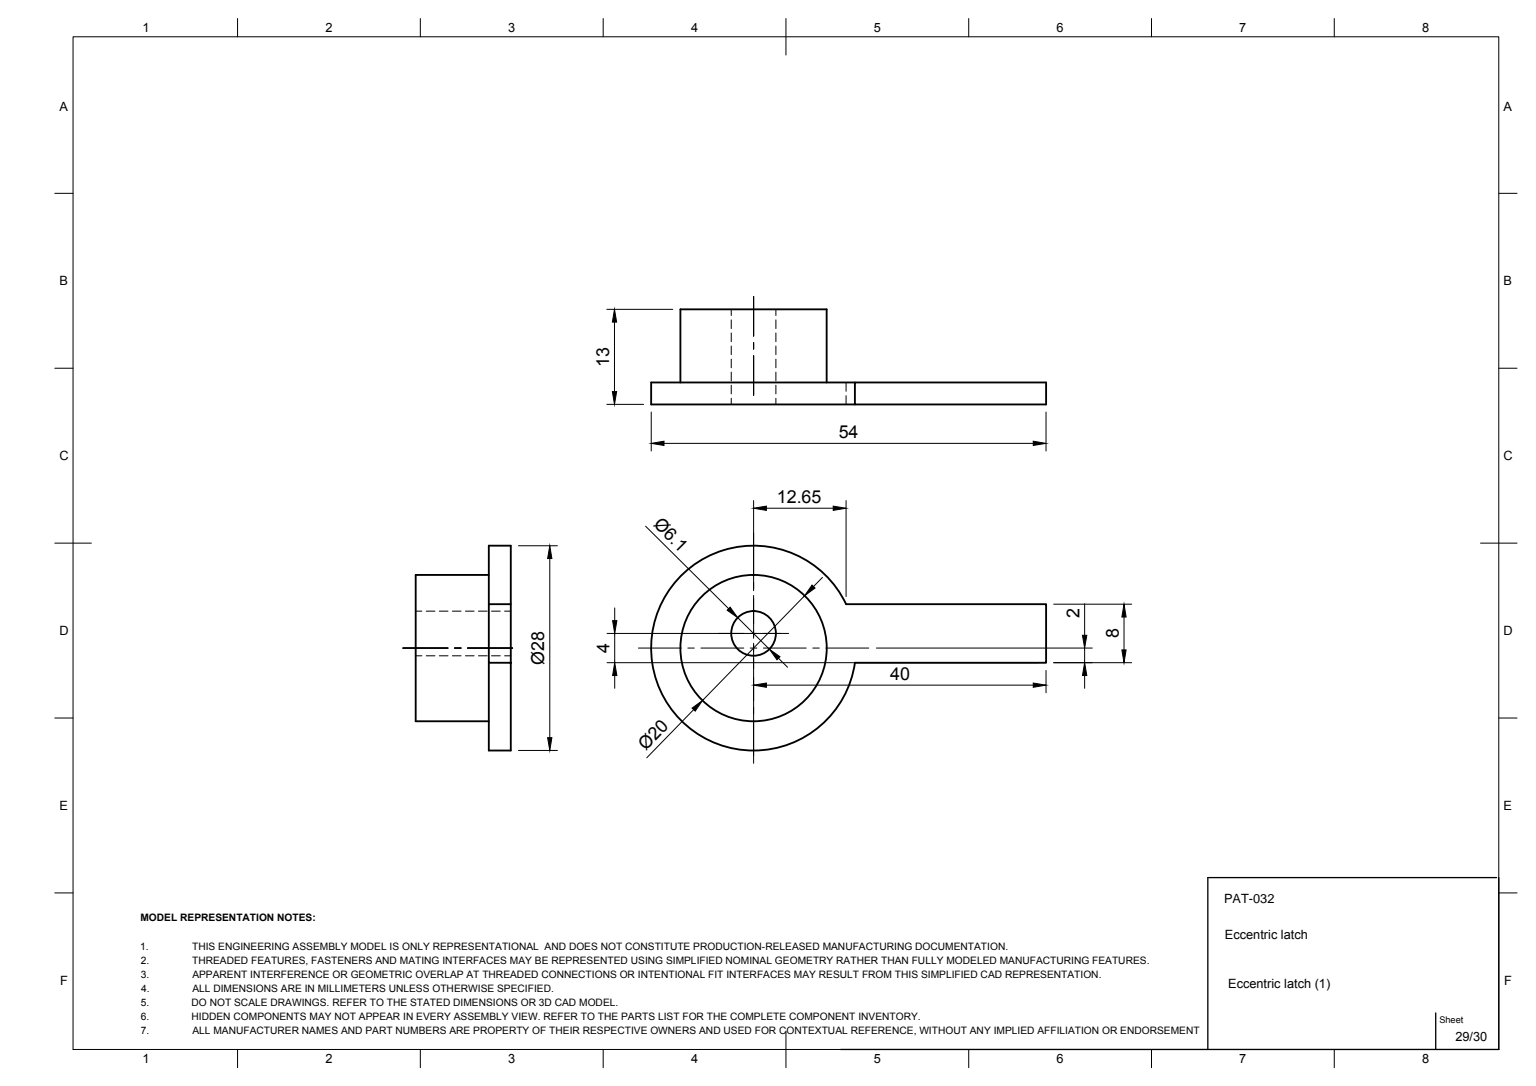
ISO-10303-21;
HEADER;
/* Generated by software containing ST-Developer
 * from STEP Tools, Inc. (www.steptools.com) 
 */

FILE_DESCRIPTION(
/* description */ ('Drill jig with bushing plate'),
/* implementation_level */ '2;1');

FILE_NAME(
/* name */ 'Eccentric latch.step',
/* time_stamp */ '2026-10-27T10:51:08-07:00',
/* author */ (''),
/* organization */ (''),
/* preprocessor_version */ 'ST-DEVELOPER v20.2',
/* originating_system */ 'Autodesk Translation Framework v15.17.0.0',
/* authorisation */ '');

FILE_SCHEMA (('AUTOMOTIVE_DESIGN { 1 0 10303 214 3 1 1 }'));
ENDSEC;

DATA;
#10=MECHANICAL_DESIGN_GEOMETRIC_PRESENTATION_REPRESENTATION('',(#245),#6638);
#197=SHAPE_REPRESENTATION_RELATIONSHIP('SRR','None',#6763,#221);
#221=ADVANCED_BREP_SHAPE_REPRESENTATION('',(#267),#6636);
#245=STYLED_ITEM('',(#6936),#267);
#267=MANIFOLD_SOLID_BREP('Body1',#3614);
#367=FACE_BOUND('',#1020,.T.);
#368=FACE_BOUND('',#1022,.T.);
#369=FACE_BOUND('',#1026,.T.);
#493=PLANE('',#4306);
#494=PLANE('',#4307);
#495=PLANE('',#4308);
#496=PLANE('',#4309);
#497=PLANE('',#4311);
#498=PLANE('',#4317);
#703=FACE_OUTER_BOUND('',#1015,.T.);
#704=FACE_OUTER_BOUND('',#1016,.T.);
#705=FACE_OUTER_BOUND('',#1017,.T.);
#706=FACE_OUTER_BOUND('',#1018,.T.);
#707=FACE_OUTER_BOUND('',#1019,.T.);
#708=FACE_OUTER_BOUND('',#1021,.T.);
#709=FACE_OUTER_BOUND('',#1023,.T.);
#710=FACE_OUTER_BOUND('',#1024,.T.);
#711=FACE_OUTER_BOUND('',#1025,.T.);
#1015=EDGE_LOOP('',(#3257,#3258,#3259,#3260));
#1016=EDGE_LOOP('',(#3261,#3262,#3263,#3264));
#1017=EDGE_LOOP('',(#3265,#3266,#3267,#3268));
#1018=EDGE_LOOP('',(#3269,#3270,#3271,#3272));
#1019=EDGE_LOOP('',(#3273,#3274,#3275,#3276));
#1020=EDGE_LOOP('',(#3277));
#1021=EDGE_LOOP('',(#3278,#3279,#3280,#3281));
#1022=EDGE_LOOP('',(#3282));
#1023=EDGE_LOOP('',(#3283,#3284,#3285,#3286));
#1024=EDGE_LOOP('',(#3287,#3288,#3289,#3290));
#1025=EDGE_LOOP('',(#3291));
#1026=EDGE_LOOP('',(#3292));
#1278=LINE('',#6532,#1539);
#1279=LINE('',#6537,#1540);
#1280=LINE('',#6539,#1541);
#1281=LINE('',#6541,#1542);
#1282=LINE('',#6542,#1543);
#1283=LINE('',#6545,#1544);
#1284=LINE('',#6547,#1545);
#1285=LINE('',#6548,#1546);
#1286=LINE('',#6552,#1547);
#1287=LINE('',#6553,#1548);
#1288=LINE('',#6554,#1549);
#1289=LINE('',#6564,#1550);
#1539=VECTOR('',#5425,0.305);
#1540=VECTOR('',#5430,1.);
#1541=VECTOR('',#5431,1.);
#1542=VECTOR('',#5432,1.);
#1543=VECTOR('',#5433,1.);
#1544=VECTOR('',#5436,1.);
#1545=VECTOR('',#5437,1.);
#1546=VECTOR('',#5438,1.);
#1547=VECTOR('',#5441,1.);
#1548=VECTOR('',#5442,1.);
#1549=VECTOR('',#5443,1.);
#1550=VECTOR('',#5458,1.);
#1712=CIRCLE('',#4304,0.305);
#1713=CIRCLE('',#4305,0.305);
#1714=CIRCLE('',#4310,1.4);
#1715=CIRCLE('',#4312,1.4);
#1716=CIRCLE('',#4313,1.);
#1717=CIRCLE('',#4316,1.);
#1992=VERTEX_POINT('',#6529);
#1993=VERTEX_POINT('',#6531);
#1994=VERTEX_POINT('',#6535);
#1995=VERTEX_POINT('',#6536);
#1996=VERTEX_POINT('',#6538);
#1997=VERTEX_POINT('',#6540);
#1998=VERTEX_POINT('',#6544);
#1999=VERTEX_POINT('',#6546);
#2000=VERTEX_POINT('',#6550);
#2001=VERTEX_POINT('',#6551);
#2002=VERTEX_POINT('',#6559);
#2003=VERTEX_POINT('',#6563);
#2416=EDGE_CURVE('',#1992,#1992,#1712,.T.);
#2417=EDGE_CURVE('',#1992,#1993,#1278,.T.);
#2418=EDGE_CURVE('',#1993,#1993,#1713,.T.);
#2419=EDGE_CURVE('',#1994,#1995,#1279,.T.);
#2420=EDGE_CURVE('',#1994,#1996,#1280,.T.);
#2421=EDGE_CURVE('',#1996,#1997,#1281,.T.);
#2422=EDGE_CURVE('',#1995,#1997,#1282,.T.);
#2423=EDGE_CURVE('',#1996,#1998,#1283,.T.);
#2424=EDGE_CURVE('',#1998,#1999,#1284,.T.);
#2425=EDGE_CURVE('',#1997,#1999,#1285,.T.);
#2426=EDGE_CURVE('',#2000,#2001,#1286,.T.);
#2427=EDGE_CURVE('',#1999,#2000,#1287,.T.);
#2428=EDGE_CURVE('',#1998,#2001,#1288,.T.);
#2429=EDGE_CURVE('',#2000,#1995,#1714,.T.);
#2430=EDGE_CURVE('',#2001,#1994,#1715,.T.);
#2431=EDGE_CURVE('',#2002,#2002,#1716,.T.);
#2432=EDGE_CURVE('',#2002,#2003,#1289,.T.);
#2433=EDGE_CURVE('',#2003,#2003,#1717,.T.);
#3257=ORIENTED_EDGE('',*,*,#2416,.F.);
#3258=ORIENTED_EDGE('',*,*,#2417,.T.);
#3259=ORIENTED_EDGE('',*,*,#2418,.F.);
#3260=ORIENTED_EDGE('',*,*,#2417,.F.);
#3261=ORIENTED_EDGE('',*,*,#2419,.F.);
#3262=ORIENTED_EDGE('',*,*,#2420,.T.);
#3263=ORIENTED_EDGE('',*,*,#2421,.T.);
#3264=ORIENTED_EDGE('',*,*,#2422,.F.);
#3265=ORIENTED_EDGE('',*,*,#2423,.T.);
#3266=ORIENTED_EDGE('',*,*,#2424,.T.);
#3267=ORIENTED_EDGE('',*,*,#2425,.F.);
#3268=ORIENTED_EDGE('',*,*,#2421,.F.);
#3269=ORIENTED_EDGE('',*,*,#2426,.F.);
#3270=ORIENTED_EDGE('',*,*,#2427,.F.);
#3271=ORIENTED_EDGE('',*,*,#2424,.F.);
#3272=ORIENTED_EDGE('',*,*,#2428,.T.);
#3273=ORIENTED_EDGE('',*,*,#2429,.T.);
#3274=ORIENTED_EDGE('',*,*,#2422,.T.);
#3275=ORIENTED_EDGE('',*,*,#2425,.T.);
#3276=ORIENTED_EDGE('',*,*,#2427,.T.);
#3277=ORIENTED_EDGE('',*,*,#2418,.T.);
#3278=ORIENTED_EDGE('',*,*,#2430,.F.);
#3279=ORIENTED_EDGE('',*,*,#2428,.F.);
#3280=ORIENTED_EDGE('',*,*,#2423,.F.);
#3281=ORIENTED_EDGE('',*,*,#2420,.F.);
#3282=ORIENTED_EDGE('',*,*,#2431,.T.);
#3283=ORIENTED_EDGE('',*,*,#2419,.T.);
#3284=ORIENTED_EDGE('',*,*,#2429,.F.);
#3285=ORIENTED_EDGE('',*,*,#2426,.T.);
#3286=ORIENTED_EDGE('',*,*,#2430,.T.);
#3287=ORIENTED_EDGE('',*,*,#2431,.F.);
#3288=ORIENTED_EDGE('',*,*,#2432,.T.);
#3289=ORIENTED_EDGE('',*,*,#2433,.T.);
#3290=ORIENTED_EDGE('',*,*,#2432,.F.);
#3291=ORIENTED_EDGE('',*,*,#2433,.F.);
#3292=ORIENTED_EDGE('',*,*,#2416,.T.);
#3372=CYLINDRICAL_SURFACE('',#4303,0.305);
#3373=CYLINDRICAL_SURFACE('',#4314,1.4);
#3374=CYLINDRICAL_SURFACE('',#4315,1.);
#3578=ADVANCED_FACE('',(#703),#3372,.F.);
#3579=ADVANCED_FACE('',(#704),#493,.T.);
#3580=ADVANCED_FACE('',(#705),#494,.T.);
#3581=ADVANCED_FACE('',(#706),#495,.T.);
#3582=ADVANCED_FACE('',(#707,#367),#496,.T.);
#3583=ADVANCED_FACE('',(#708,#368),#497,.F.);
#3584=ADVANCED_FACE('',(#709),#3373,.T.);
#3585=ADVANCED_FACE('',(#710),#3374,.T.);
#3586=ADVANCED_FACE('',(#711,#369),#498,.F.);
#3614=CLOSED_SHELL('',(#3578,#3579,#3580,#3581,#3582,#3583,#3584,#3585,
#3586));
#4302=AXIS2_PLACEMENT_3D('',#6527,#5419,#5420);
#4303=AXIS2_PLACEMENT_3D('',#6528,#5421,#5422);
#4304=AXIS2_PLACEMENT_3D('',#6530,#5423,#5424);
#4305=AXIS2_PLACEMENT_3D('',#6533,#5426,#5427);
#4306=AXIS2_PLACEMENT_3D('',#6534,#5428,#5429);
#4307=AXIS2_PLACEMENT_3D('',#6543,#5434,#5435);
#4308=AXIS2_PLACEMENT_3D('',#6549,#5439,#5440);
#4309=AXIS2_PLACEMENT_3D('',#6555,#5444,#5445);
#4310=AXIS2_PLACEMENT_3D('',#6556,#5446,#5447);
#4311=AXIS2_PLACEMENT_3D('',#6557,#5448,#5449);
#4312=AXIS2_PLACEMENT_3D('',#6558,#5450,#5451);
#4313=AXIS2_PLACEMENT_3D('',#6560,#5452,#5453);
#4314=AXIS2_PLACEMENT_3D('',#6561,#5454,#5455);
#4315=AXIS2_PLACEMENT_3D('',#6562,#5456,#5457);
#4316=AXIS2_PLACEMENT_3D('',#6565,#5459,#5460);
#4317=AXIS2_PLACEMENT_3D('',#6566,#5461,#5462);
#5419=DIRECTION('axis',(0.,0.,1.));
#5420=DIRECTION('refdir',(1.,0.,0.));
#5421=DIRECTION('center_axis',(0.,0.,1.));
#5422=DIRECTION('ref_axis',(1.,0.,0.));
#5423=DIRECTION('center_axis',(0.,0.,1.));
#5424=DIRECTION('ref_axis',(1.,0.,0.));
#5425=DIRECTION('',(0.,0.,1.));
#5426=DIRECTION('center_axis',(0.,0.,-1.));
#5427=DIRECTION('ref_axis',(1.,0.,0.));
#5428=DIRECTION('center_axis',(1.,0.,0.));
#5429=DIRECTION('ref_axis',(0.,1.,0.));
#5430=DIRECTION('',(0.,0.,1.));
#5431=DIRECTION('',(0.,1.,0.));
#5432=DIRECTION('',(0.,0.,1.));
#5433=DIRECTION('',(0.,1.,0.));
#5434=DIRECTION('center_axis',(0.,1.,0.));
#5435=DIRECTION('ref_axis',(-1.,0.,0.));
#5436=DIRECTION('',(-1.,0.,0.));
#5437=DIRECTION('',(0.,0.,1.));
#5438=DIRECTION('',(-1.,0.,0.));
#5439=DIRECTION('center_axis',(-1.,0.,0.));
#5440=DIRECTION('ref_axis',(0.,-1.,0.));
#5441=DIRECTION('',(0.,0.,-1.));
#5442=DIRECTION('',(0.,-1.,0.));
#5443=DIRECTION('',(0.,-1.,0.));
#5444=DIRECTION('center_axis',(0.,0.,1.));
#5445=DIRECTION('ref_axis',(1.,0.,0.));
#5446=DIRECTION('center_axis',(0.,0.,1.));
#5447=DIRECTION('ref_axis',(1.,0.,0.));
#5448=DIRECTION('center_axis',(0.,0.,1.));
#5449=DIRECTION('ref_axis',(1.,0.,0.));
#5450=DIRECTION('center_axis',(0.,0.,1.));
#5451=DIRECTION('ref_axis',(1.,0.,0.));
#5452=DIRECTION('center_axis',(0.,0.,1.));
#5453=DIRECTION('ref_axis',(1.,0.,0.));
#5454=DIRECTION('center_axis',(0.,0.,1.));
#5455=DIRECTION('ref_axis',(-0.149222317351604,-0.988803671111823,0.));
#5456=DIRECTION('center_axis',(0.,0.,1.));
#5457=DIRECTION('ref_axis',(1.,0.,0.));
#5458=DIRECTION('',(0.,0.,-1.));
#5459=DIRECTION('center_axis',(0.,0.,1.));
#5460=DIRECTION('ref_axis',(1.,0.,0.));
#5461=DIRECTION('center_axis',(0.,0.,1.));
#5462=DIRECTION('ref_axis',(1.,0.,0.));
#6527=CARTESIAN_POINT('',(0.,0.,0.));
#6528=CARTESIAN_POINT('Origin',(9.2,3.5,3.4));
#6529=CARTESIAN_POINT('',(8.895,3.5,3.5));
#6530=CARTESIAN_POINT('Origin',(9.2,3.5,3.5));
#6531=CARTESIAN_POINT('',(8.895,3.5,4.8));
#6532=CARTESIAN_POINT('',(8.895,3.5,3.4));
#6533=CARTESIAN_POINT('Origin',(9.2,3.5,4.8));
#6534=CARTESIAN_POINT('Origin',(9.6,3.5,4.5));
#6535=CARTESIAN_POINT('',(9.6,4.76491106406735,4.5));
#6536=CARTESIAN_POINT('',(9.6,4.76491106406735,4.8));
#6537=CARTESIAN_POINT('',(9.6,4.76491106406735,4.5));
#6538=CARTESIAN_POINT('',(9.6,7.5,4.5));
#6539=CARTESIAN_POINT('',(9.6,3.5,4.5));
#6540=CARTESIAN_POINT('',(9.6,7.5,4.8));
#6541=CARTESIAN_POINT('',(9.6,7.5,4.5));
#6542=CARTESIAN_POINT('',(9.6,3.5,4.8));
#6543=CARTESIAN_POINT('Origin',(9.6,7.5,4.5));
#6544=CARTESIAN_POINT('',(8.8,7.5,4.5));
#6545=CARTESIAN_POINT('',(9.6,7.5,4.5));
#6546=CARTESIAN_POINT('',(8.8,7.5,4.8));
#6547=CARTESIAN_POINT('',(8.8,7.5,4.5));
#6548=CARTESIAN_POINT('',(9.6,7.5,4.8));
#6549=CARTESIAN_POINT('Origin',(8.8,7.5,4.5));
#6550=CARTESIAN_POINT('',(8.8,4.8856406460551,4.8));
#6551=CARTESIAN_POINT('',(8.8,4.8856406460551,4.5));
#6552=CARTESIAN_POINT('',(8.8,4.8856406460551,4.5));
#6553=CARTESIAN_POINT('',(8.8,7.5,4.8));
#6554=CARTESIAN_POINT('',(8.8,7.5,4.5));
#6555=CARTESIAN_POINT('Origin',(9.,3.5,4.8));
#6556=CARTESIAN_POINT('Origin',(9.,3.5,4.8));
#6557=CARTESIAN_POINT('Origin',(9.,3.5,4.5));
#6558=CARTESIAN_POINT('Origin',(9.,3.5,4.5));
#6559=CARTESIAN_POINT('',(8.,3.5,4.5));
#6560=CARTESIAN_POINT('Origin',(9.,3.5,4.5));
#6561=CARTESIAN_POINT('Origin',(9.,3.5,4.5));
#6562=CARTESIAN_POINT('Origin',(9.,3.5,3.5));
#6563=CARTESIAN_POINT('',(8.,3.5,3.5));
#6564=CARTESIAN_POINT('',(8.,3.5,3.5));
#6565=CARTESIAN_POINT('Origin',(9.,3.5,3.5));
#6566=CARTESIAN_POINT('Origin',(9.,3.5,3.5));
#6607=UNCERTAINTY_MEASURE_WITH_UNIT(LENGTH_MEASURE(0.001),#6639,
'DISTANCE_ACCURACY_VALUE',
'Maximum model space distance between geometric entities at asserted c
onnectivities');
#6609=UNCERTAINTY_MEASURE_WITH_UNIT(LENGTH_MEASURE(0.001),#6639,
'DISTANCE_ACCURACY_VALUE',
'Maximum model space distance between geometric entities at asserted c
onnectivities');
#6636=(
GEOMETRIC_REPRESENTATION_CONTEXT(3)
GLOBAL_UNCERTAINTY_ASSIGNED_CONTEXT((#6607))
GLOBAL_UNIT_ASSIGNED_CONTEXT((#6639,#6641,#6642))
REPRESENTATION_CONTEXT('','3D')
);
#6638=(
GEOMETRIC_REPRESENTATION_CONTEXT(3)
GLOBAL_UNCERTAINTY_ASSIGNED_CONTEXT((#6609))
GLOBAL_UNIT_ASSIGNED_CONTEXT((#6639,#6641,#6642))
REPRESENTATION_CONTEXT('','3D')
);
#6639=(
LENGTH_UNIT()
NAMED_UNIT(*)
SI_UNIT(.CENTI.,.METRE.)
);
#6641=(
NAMED_UNIT(*)
PLANE_ANGLE_UNIT()
SI_UNIT($,.RADIAN.)
);
#6642=(
NAMED_UNIT(*)
SI_UNIT($,.STERADIAN.)
SOLID_ANGLE_UNIT()
);
#6669=SHAPE_DEFINITION_REPRESENTATION(#6730,#6763);
#6730=PRODUCT_DEFINITION_SHAPE('',$,#6792);
#6763=SHAPE_REPRESENTATION('',(#4302),#6636);
#6765=PRODUCT_DEFINITION_CONTEXT('part definition',#6851,'design');
#6792=PRODUCT_DEFINITION('Eccentric latch','Eccentric latch',#6820,#6765);
#6820=PRODUCT_DEFINITION_FORMATION('',$,#6879);
#6851=APPLICATION_CONTEXT(
'Core Data for Automotive Mechanical Design Process');
#6852=PRODUCT_CONTEXT('part definition',#6851,'mechanical');
#6879=PRODUCT('Eccentric latch','Eccentric latch','Eccentric latch',(#6852));
#6930=COLOUR_RGB('Sky Blue',0.24,0.69,0.87);
#6931=FILL_AREA_STYLE_COLOUR('',#6930);
#6932=FILL_AREA_STYLE('',(#6931));
#6933=SURFACE_STYLE_FILL_AREA(#6932);
#6934=SURFACE_SIDE_STYLE('',(#6933));
#6935=SURFACE_STYLE_USAGE(.BOTH.,#6934);
#6936=PRESENTATION_STYLE_ASSIGNMENT((#6935));
ENDSEC;
END-ISO-10303-21;
